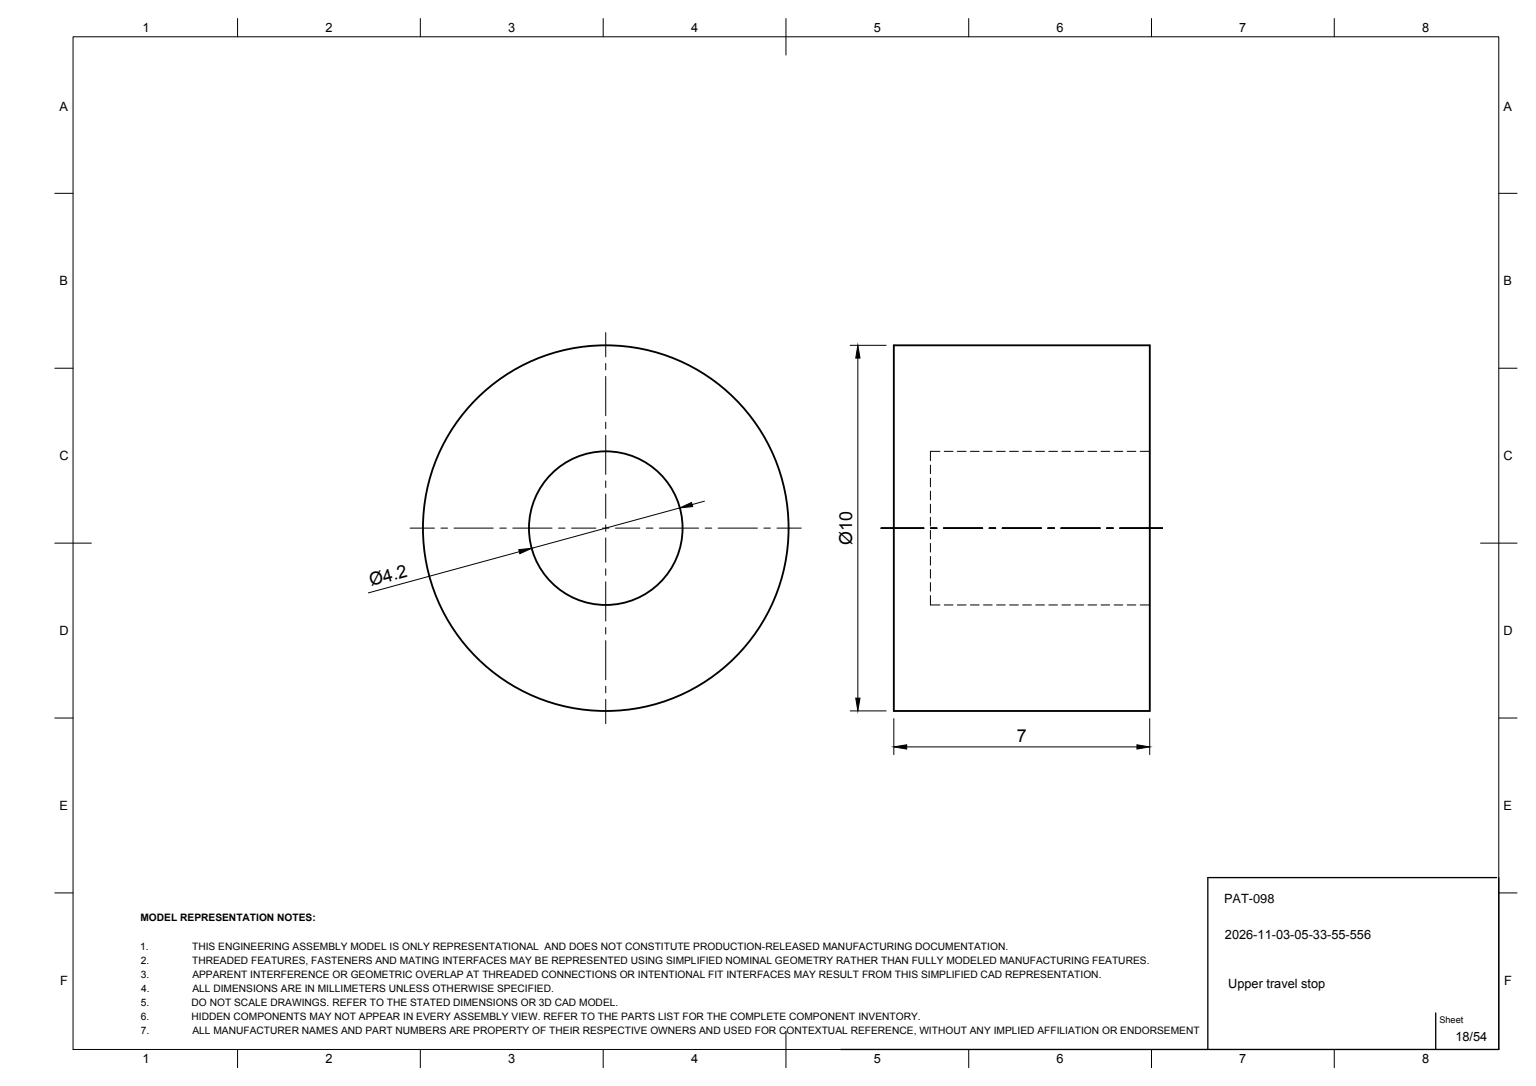
ISO-10303-21;
HEADER;
/* Generated by software containing ST-Developer
 * from STEP Tools, Inc. (www.steptools.com) 
 */

FILE_DESCRIPTION(
/* description */ ('Spring compression tester'),
/* implementation_level */ '2;1');

FILE_NAME(
/* name */ 'Upper travel stop.step',
/* time_stamp */ '2026-10-28T03:24:11-07:00',
/* author */ (''),
/* organization */ (''),
/* preprocessor_version */ 'ST-DEVELOPER v20.2',
/* originating_system */ 'Autodesk Translation Framework v15.17.0.0',
/* authorisation */ '');

FILE_SCHEMA (('AUTOMOTIVE_DESIGN { 1 0 10303 214 3 1 1 }'));
ENDSEC;

DATA;
#10=MECHANICAL_DESIGN_GEOMETRIC_PRESENTATION_REPRESENTATION('',(#1119),#43521);
#999=SHAPE_REPRESENTATION_RELATIONSHIP('SRR','None',#43811,#1059);
#1059=ADVANCED_BREP_SHAPE_REPRESENTATION('',(#1194),#43471);
#1119=STYLED_ITEM('',(#44216),#1194);
#1194=MANIFOLD_SOLID_BREP('Body1',#18556);
#1395=FACE_BOUND('',#3588,.T.);
#1713=PLANE('',#19722);
#1714=PLANE('',#19726);
#1715=PLANE('',#19727);
#2389=FACE_OUTER_BOUND('',#3584,.T.);
#2390=FACE_OUTER_BOUND('',#3585,.T.);
#2391=FACE_OUTER_BOUND('',#3586,.T.);
#2392=FACE_OUTER_BOUND('',#3587,.T.);
#2393=FACE_OUTER_BOUND('',#3589,.T.);
#3584=EDGE_LOOP('',(#13195,#13196,#13197,#13198));
#3585=EDGE_LOOP('',(#13199));
#3586=EDGE_LOOP('',(#13200,#13201,#13202,#13203));
#3587=EDGE_LOOP('',(#13204));
#3588=EDGE_LOOP('',(#13205));
#3589=EDGE_LOOP('',(#13206));
#4897=LINE('',#27508,#6329);
#4898=LINE('',#27515,#6330);
#6329=VECTOR('',#22361,0.21);
#6330=VECTOR('',#22370,0.5);
#7668=CIRCLE('',#19720,0.21);
#7669=CIRCLE('',#19721,0.21);
#7670=CIRCLE('',#19724,0.5);
#7671=CIRCLE('',#19725,0.5);
#8462=VERTEX_POINT('',#27505);
#8463=VERTEX_POINT('',#27507);
#8464=VERTEX_POINT('',#27512);
#8465=VERTEX_POINT('',#27514);
#10262=EDGE_CURVE('',#8462,#8462,#7668,.T.);
#10263=EDGE_CURVE('',#8462,#8463,#4897,.T.);
#10264=EDGE_CURVE('',#8463,#8463,#7669,.T.);
#10265=EDGE_CURVE('',#8464,#8464,#7670,.T.);
#10266=EDGE_CURVE('',#8464,#8465,#4898,.T.);
#10267=EDGE_CURVE('',#8465,#8465,#7671,.T.);
#13195=ORIENTED_EDGE('',*,*,#10262,.F.);
#13196=ORIENTED_EDGE('',*,*,#10263,.T.);
#13197=ORIENTED_EDGE('',*,*,#10264,.F.);
#13198=ORIENTED_EDGE('',*,*,#10263,.F.);
#13199=ORIENTED_EDGE('',*,*,#10262,.T.);
#13200=ORIENTED_EDGE('',*,*,#10265,.F.);
#13201=ORIENTED_EDGE('',*,*,#10266,.T.);
#13202=ORIENTED_EDGE('',*,*,#10267,.T.);
#13203=ORIENTED_EDGE('',*,*,#10266,.F.);
#13204=ORIENTED_EDGE('',*,*,#10265,.T.);
#13205=ORIENTED_EDGE('',*,*,#10264,.T.);
#13206=ORIENTED_EDGE('',*,*,#10267,.F.);
#17200=CYLINDRICAL_SURFACE('',#19719,0.21);
#17201=CYLINDRICAL_SURFACE('',#19723,0.5);
#17713=ADVANCED_FACE('',(#2389),#17200,.F.);
#17714=ADVANCED_FACE('',(#2390),#1713,.T.);
#17715=ADVANCED_FACE('',(#2391),#17201,.T.);
#17716=ADVANCED_FACE('',(#2392,#1395),#1714,.T.);
#17717=ADVANCED_FACE('',(#2393),#1715,.F.);
#18556=CLOSED_SHELL('',(#17713,#17714,#17715,#17716,#17717));
#19718=AXIS2_PLACEMENT_3D('',#27503,#22355,#22356);
#19719=AXIS2_PLACEMENT_3D('',#27504,#22357,#22358);
#19720=AXIS2_PLACEMENT_3D('',#27506,#22359,#22360);
#19721=AXIS2_PLACEMENT_3D('',#27509,#22362,#22363);
#19722=AXIS2_PLACEMENT_3D('',#27510,#22364,#22365);
#19723=AXIS2_PLACEMENT_3D('',#27511,#22366,#22367);
#19724=AXIS2_PLACEMENT_3D('',#27513,#22368,#22369);
#19725=AXIS2_PLACEMENT_3D('',#27516,#22371,#22372);
#19726=AXIS2_PLACEMENT_3D('',#27517,#22373,#22374);
#19727=AXIS2_PLACEMENT_3D('',#27518,#22375,#22376);
#22355=DIRECTION('axis',(0.,0.,1.));
#22356=DIRECTION('refdir',(1.,0.,0.));
#22357=DIRECTION('center_axis',(0.,0.,1.));
#22358=DIRECTION('ref_axis',(1.,0.,0.));
#22359=DIRECTION('center_axis',(0.,0.,1.));
#22360=DIRECTION('ref_axis',(1.,0.,0.));
#22361=DIRECTION('',(0.,0.,1.));
#22362=DIRECTION('center_axis',(0.,0.,-1.));
#22363=DIRECTION('ref_axis',(1.,0.,0.));
#22364=DIRECTION('center_axis',(0.,0.,1.));
#22365=DIRECTION('ref_axis',(1.,0.,0.));
#22366=DIRECTION('center_axis',(0.,0.,1.));
#22367=DIRECTION('ref_axis',(1.,0.,0.));
#22368=DIRECTION('center_axis',(0.,0.,1.));
#22369=DIRECTION('ref_axis',(1.,0.,0.));
#22370=DIRECTION('',(0.,0.,-1.));
#22371=DIRECTION('center_axis',(0.,0.,1.));
#22372=DIRECTION('ref_axis',(1.,0.,0.));
#22373=DIRECTION('center_axis',(0.,0.,1.));
#22374=DIRECTION('ref_axis',(1.,0.,0.));
#22375=DIRECTION('center_axis',(0.,0.,1.));
#22376=DIRECTION('ref_axis',(1.,0.,0.));
#27503=CARTESIAN_POINT('',(0.,0.,0.));
#27504=CARTESIAN_POINT('Origin',(-6.,5.,22.4));
#27505=CARTESIAN_POINT('',(-6.21,5.,22.4));
#27506=CARTESIAN_POINT('Origin',(-6.,5.,22.4));
#27507=CARTESIAN_POINT('',(-6.21,5.,23.));
#27508=CARTESIAN_POINT('',(-6.21,5.,22.4));
#27509=CARTESIAN_POINT('Origin',(-6.,5.,23.));
#27510=CARTESIAN_POINT('Origin',(-6.,5.,22.4));
#27511=CARTESIAN_POINT('Origin',(-6.,5.,22.3));
#27512=CARTESIAN_POINT('',(-6.5,5.,23.));
#27513=CARTESIAN_POINT('Origin',(-6.,5.,23.));
#27514=CARTESIAN_POINT('',(-6.5,5.,22.3));
#27515=CARTESIAN_POINT('',(-6.5,5.,22.3));
#27516=CARTESIAN_POINT('Origin',(-6.,5.,22.3));
#27517=CARTESIAN_POINT('Origin',(-6.,5.,23.));
#27518=CARTESIAN_POINT('Origin',(-6.,5.,22.3));
#43403=UNCERTAINTY_MEASURE_WITH_UNIT(LENGTH_MEASURE(0.001),#43522,
'DISTANCE_ACCURACY_VALUE',
'Maximum model space distance between geometric entities at asserted c
onnectivities');
#43453=UNCERTAINTY_MEASURE_WITH_UNIT(LENGTH_MEASURE(0.001),#43522,
'DISTANCE_ACCURACY_VALUE',
'Maximum model space distance between geometric entities at asserted c
onnectivities');
#43471=(
GEOMETRIC_REPRESENTATION_CONTEXT(3)
GLOBAL_UNCERTAINTY_ASSIGNED_CONTEXT((#43403))
GLOBAL_UNIT_ASSIGNED_CONTEXT((#43522,#43524,#43525))
REPRESENTATION_CONTEXT('','3D')
);
#43521=(
GEOMETRIC_REPRESENTATION_CONTEXT(3)
GLOBAL_UNCERTAINTY_ASSIGNED_CONTEXT((#43453))
GLOBAL_UNIT_ASSIGNED_CONTEXT((#43522,#43524,#43525))
REPRESENTATION_CONTEXT('','3D')
);
#43522=(
LENGTH_UNIT()
NAMED_UNIT(*)
SI_UNIT(.CENTI.,.METRE.)
);
#43524=(
NAMED_UNIT(*)
PLANE_ANGLE_UNIT()
SI_UNIT($,.RADIAN.)
);
#43525=(
NAMED_UNIT(*)
SI_UNIT($,.STERADIAN.)
SOLID_ANGLE_UNIT()
);
#43543=SHAPE_DEFINITION_REPRESENTATION(#43610,#43811);
#43610=PRODUCT_DEFINITION_SHAPE('',$,#43879);
#43811=SHAPE_REPRESENTATION('',(#19718),#43471);
#43861=PRODUCT_DEFINITION_CONTEXT('part definition',#44064,'design');
#43879=PRODUCT_DEFINITION('Upper travel stop','Upper travel stop',#43946,
#43861);
#43946=PRODUCT_DEFINITION_FORMATION('',$,#44083);
#44064=APPLICATION_CONTEXT(
'Core Data for Automotive Mechanical Design Process');
#44065=PRODUCT_CONTEXT('part definition',#44064,'mechanical');
#44083=PRODUCT('Upper travel stop','Upper travel stop',
'Upper travel stop',(#44065));
#44210=COLOUR_RGB('Off White',0.89,0.88,0.83);
#44211=FILL_AREA_STYLE_COLOUR('',#44210);
#44212=FILL_AREA_STYLE('',(#44211));
#44213=SURFACE_STYLE_FILL_AREA(#44212);
#44214=SURFACE_SIDE_STYLE('',(#44213));
#44215=SURFACE_STYLE_USAGE(.BOTH.,#44214);
#44216=PRESENTATION_STYLE_ASSIGNMENT((#44215));
ENDSEC;
END-ISO-10303-21;
